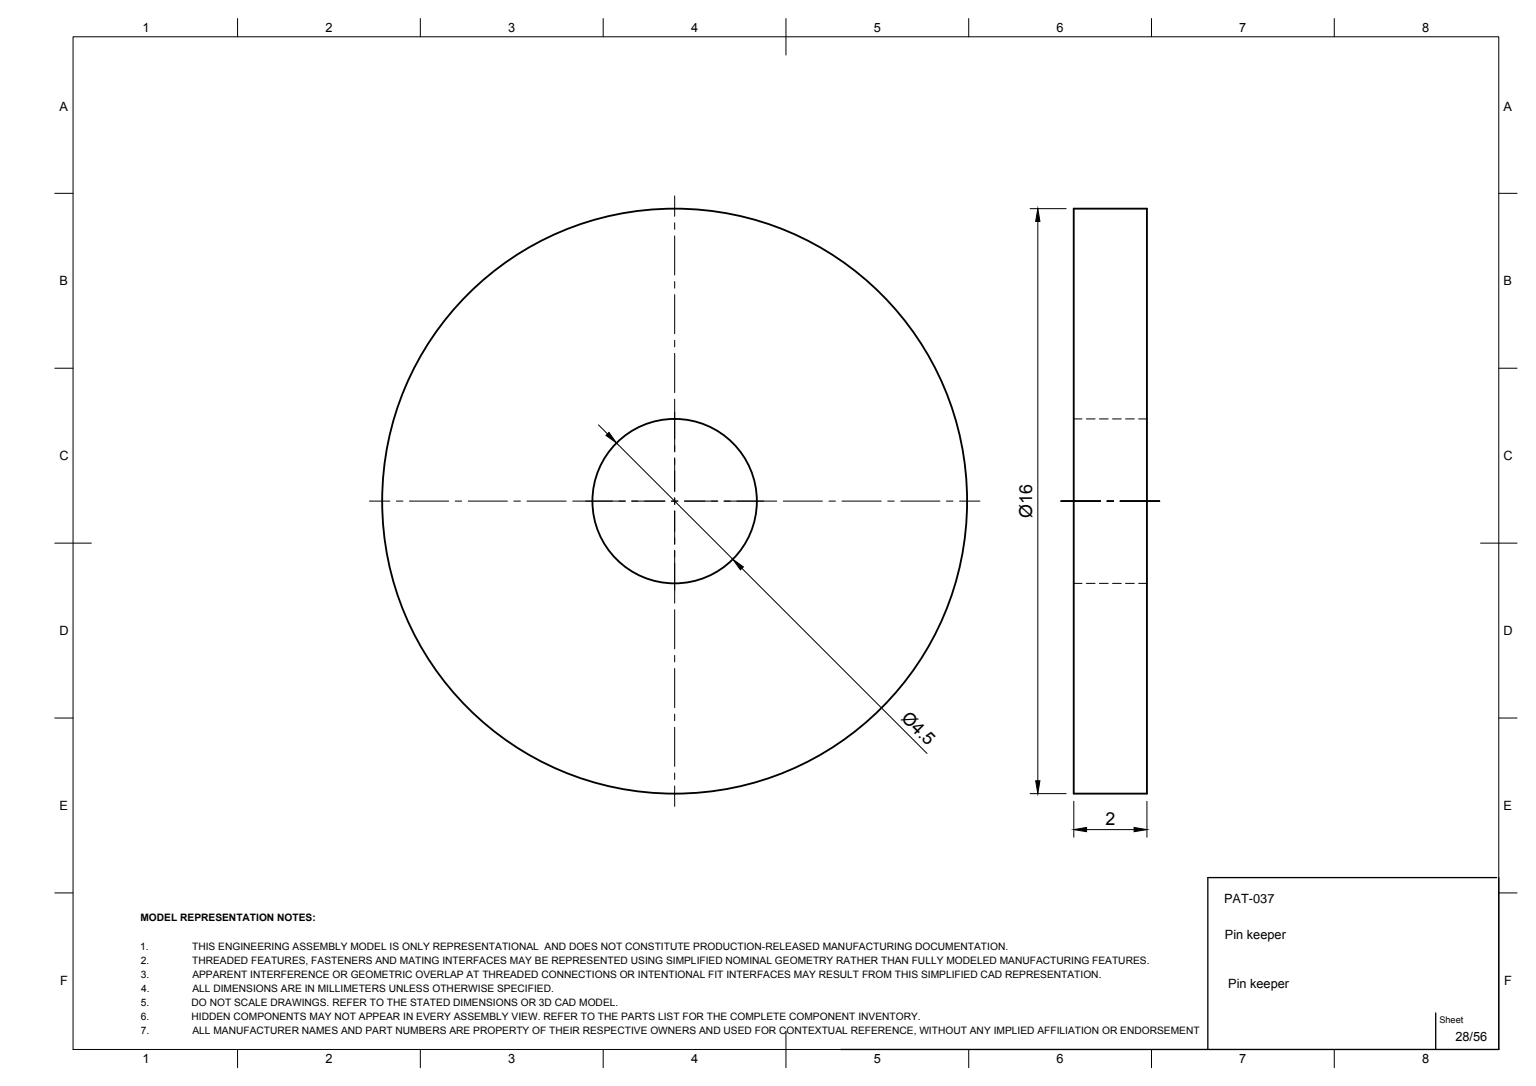
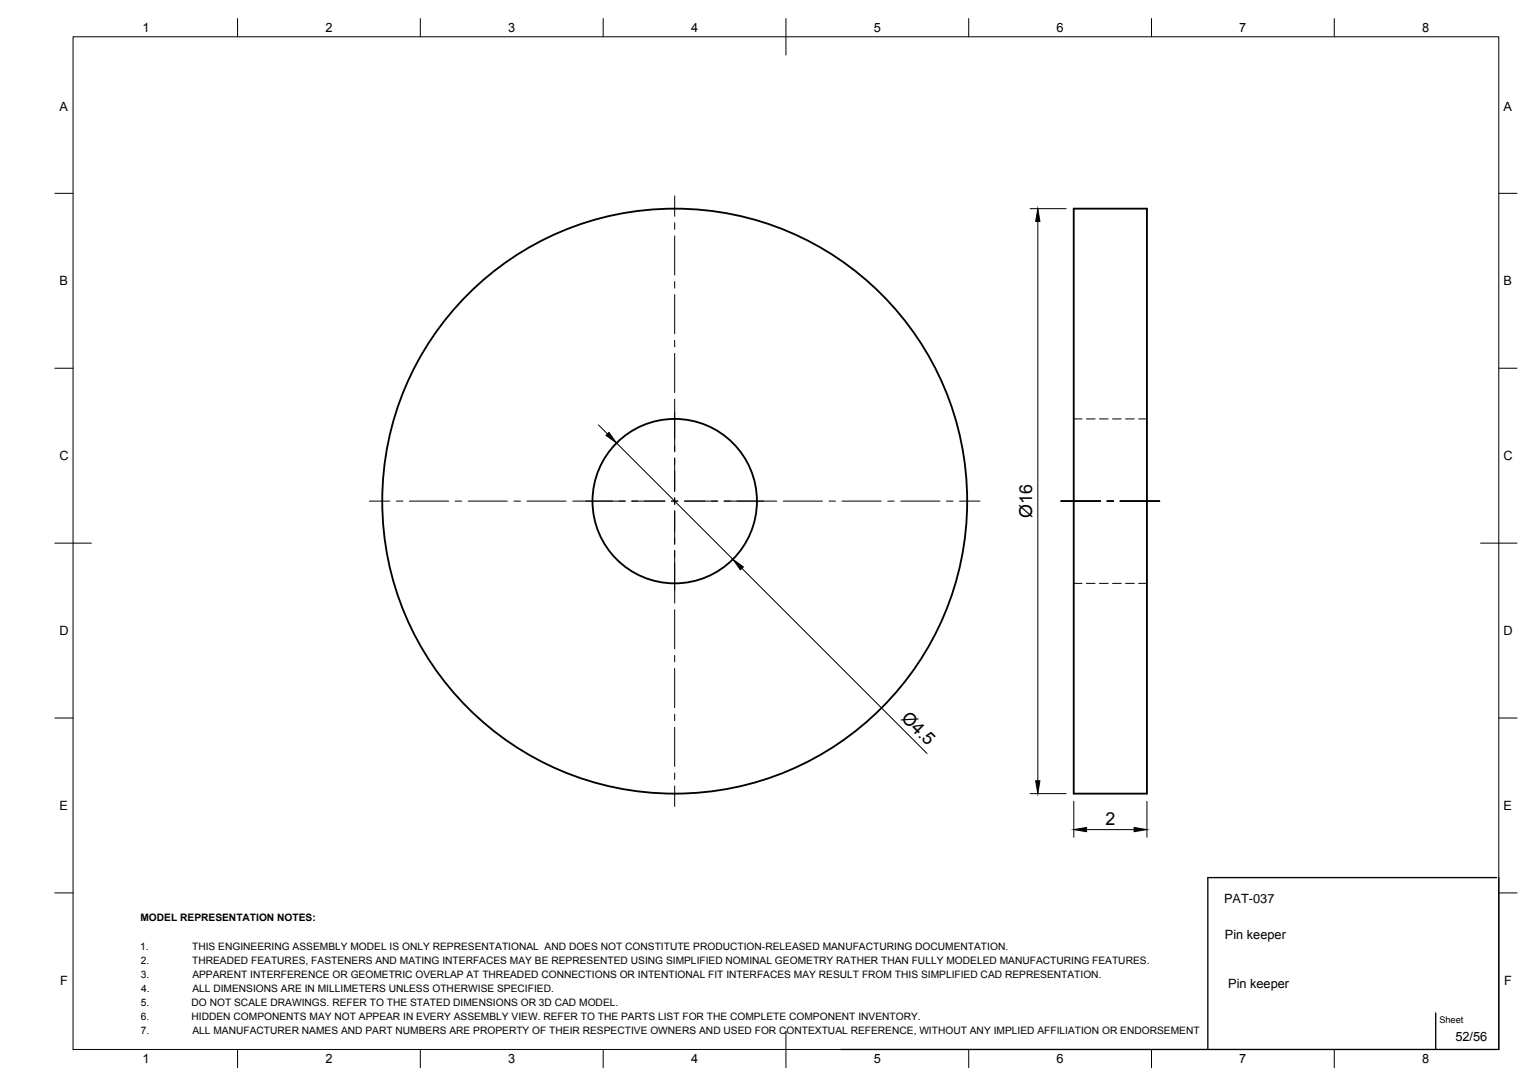
ISO-10303-21;
HEADER;
/* Generated by software containing ST-Developer
 * from STEP Tools, Inc. (www.steptools.com) 
 */

FILE_DESCRIPTION(
/* description */ ('Flywheel Crank-Slider'),
/* implementation_level */ '2;1');

FILE_NAME(
/* name */ 'Pin keeper.step',
/* time_stamp */ '2026-10-28T03:23:13-07:00',
/* author */ (''),
/* organization */ (''),
/* preprocessor_version */ 'ST-DEVELOPER v20.2',
/* originating_system */ 'Autodesk Translation Framework v15.17.0.0',
/* authorisation */ '');

FILE_SCHEMA (('AUTOMOTIVE_DESIGN { 1 0 10303 214 3 1 1 }'));
ENDSEC;

DATA;
#10=MECHANICAL_DESIGN_GEOMETRIC_PRESENTATION_REPRESENTATION('',(#698),#17322);
#593=SHAPE_REPRESENTATION_RELATIONSHIP('SRR','None',#17591,#645);
#645=ADVANCED_BREP_SHAPE_REPRESENTATION('',(#755),#17295);
#698=STYLED_ITEM('',(#17931),#755);
#755=MANIFOLD_SOLID_BREP('Body1',#9080);
#928=FACE_BOUND('',#2333,.T.);
#929=FACE_BOUND('',#2335,.T.);
#1209=PLANE('',#10309);
#1210=PLANE('',#10310);
#1652=FACE_OUTER_BOUND('',#2330,.T.);
#1653=FACE_OUTER_BOUND('',#2331,.T.);
#1654=FACE_OUTER_BOUND('',#2332,.T.);
#1655=FACE_OUTER_BOUND('',#2334,.T.);
#2330=EDGE_LOOP('',(#7504,#7505,#7506,#7507));
#2331=EDGE_LOOP('',(#7508,#7509,#7510,#7511));
#2332=EDGE_LOOP('',(#7512));
#2333=EDGE_LOOP('',(#7513));
#2334=EDGE_LOOP('',(#7514));
#2335=EDGE_LOOP('',(#7515));
#3021=LINE('',#15833,#3632);
#3022=LINE('',#15839,#3633);
#3632=VECTOR('',#12475,0.225);
#3633=VECTOR('',#12482,0.8);
#4088=CIRCLE('',#10304,0.225);
#4089=CIRCLE('',#10305,0.225);
#4090=CIRCLE('',#10307,0.8);
#4091=CIRCLE('',#10308,0.8);
#4735=VERTEX_POINT('',#15830);
#4736=VERTEX_POINT('',#15832);
#4737=VERTEX_POINT('',#15836);
#4738=VERTEX_POINT('',#15838);
#5709=EDGE_CURVE('',#4735,#4735,#4088,.T.);
#5710=EDGE_CURVE('',#4735,#4736,#3021,.T.);
#5711=EDGE_CURVE('',#4736,#4736,#4089,.T.);
#5712=EDGE_CURVE('',#4737,#4737,#4090,.T.);
#5713=EDGE_CURVE('',#4737,#4738,#3022,.T.);
#5714=EDGE_CURVE('',#4738,#4738,#4091,.T.);
#7504=ORIENTED_EDGE('',*,*,#5709,.F.);
#7505=ORIENTED_EDGE('',*,*,#5710,.T.);
#7506=ORIENTED_EDGE('',*,*,#5711,.T.);
#7507=ORIENTED_EDGE('',*,*,#5710,.F.);
#7508=ORIENTED_EDGE('',*,*,#5712,.F.);
#7509=ORIENTED_EDGE('',*,*,#5713,.T.);
#7510=ORIENTED_EDGE('',*,*,#5714,.T.);
#7511=ORIENTED_EDGE('',*,*,#5713,.F.);
#7512=ORIENTED_EDGE('',*,*,#5712,.T.);
#7513=ORIENTED_EDGE('',*,*,#5709,.T.);
#7514=ORIENTED_EDGE('',*,*,#5714,.F.);
#7515=ORIENTED_EDGE('',*,*,#5711,.F.);
#8446=CYLINDRICAL_SURFACE('',#10303,0.225);
#8447=CYLINDRICAL_SURFACE('',#10306,0.8);
#8843=ADVANCED_FACE('',(#1652),#8446,.F.);
#8844=ADVANCED_FACE('',(#1653),#8447,.T.);
#8845=ADVANCED_FACE('',(#1654,#928),#1209,.T.);
#8846=ADVANCED_FACE('',(#1655,#929),#1210,.F.);
#9080=CLOSED_SHELL('',(#8843,#8844,#8845,#8846));
#10302=AXIS2_PLACEMENT_3D('',#15828,#12469,#12470);
#10303=AXIS2_PLACEMENT_3D('',#15829,#12471,#12472);
#10304=AXIS2_PLACEMENT_3D('',#15831,#12473,#12474);
#10305=AXIS2_PLACEMENT_3D('',#15834,#12476,#12477);
#10306=AXIS2_PLACEMENT_3D('',#15835,#12478,#12479);
#10307=AXIS2_PLACEMENT_3D('',#15837,#12480,#12481);
#10308=AXIS2_PLACEMENT_3D('',#15840,#12483,#12484);
#10309=AXIS2_PLACEMENT_3D('',#15841,#12485,#12486);
#10310=AXIS2_PLACEMENT_3D('',#15842,#12487,#12488);
#12469=DIRECTION('axis',(0.,0.,1.));
#12470=DIRECTION('refdir',(1.,0.,0.));
#12471=DIRECTION('center_axis',(0.,1.,0.));
#12472=DIRECTION('ref_axis',(1.,0.,0.));
#12473=DIRECTION('center_axis',(0.,-1.,0.));
#12474=DIRECTION('ref_axis',(1.,0.,0.));
#12475=DIRECTION('',(0.,-1.,0.));
#12476=DIRECTION('center_axis',(0.,-1.,0.));
#12477=DIRECTION('ref_axis',(1.,0.,0.));
#12478=DIRECTION('center_axis',(0.,1.,0.));
#12479=DIRECTION('ref_axis',(1.,0.,0.));
#12480=DIRECTION('center_axis',(0.,1.,0.));
#12481=DIRECTION('ref_axis',(1.,0.,0.));
#12482=DIRECTION('',(0.,-1.,0.));
#12483=DIRECTION('center_axis',(0.,1.,0.));
#12484=DIRECTION('ref_axis',(1.,0.,0.));
#12485=DIRECTION('center_axis',(0.,1.,0.));
#12486=DIRECTION('ref_axis',(1.,0.,0.));
#12487=DIRECTION('center_axis',(0.,1.,0.));
#12488=DIRECTION('ref_axis',(1.,0.,0.));
#15828=CARTESIAN_POINT('',(0.,0.,0.));
#15829=CARTESIAN_POINT('Origin',(2.,3.8,10.));
#15830=CARTESIAN_POINT('',(1.775,4.,10.));
#15831=CARTESIAN_POINT('Origin',(2.,4.,10.));
#15832=CARTESIAN_POINT('',(1.775,3.8,10.));
#15833=CARTESIAN_POINT('',(1.775,3.8,10.));
#15834=CARTESIAN_POINT('Origin',(2.,3.8,10.));
#15835=CARTESIAN_POINT('Origin',(2.,3.8,10.));
#15836=CARTESIAN_POINT('',(1.2,4.,10.));
#15837=CARTESIAN_POINT('Origin',(2.,4.,10.));
#15838=CARTESIAN_POINT('',(1.2,3.8,10.));
#15839=CARTESIAN_POINT('',(1.2,3.8,10.));
#15840=CARTESIAN_POINT('Origin',(2.,3.8,10.));
#15841=CARTESIAN_POINT('Origin',(2.,4.,10.));
#15842=CARTESIAN_POINT('Origin',(2.,3.8,10.));
#17234=UNCERTAINTY_MEASURE_WITH_UNIT(LENGTH_MEASURE(0.001),#17323,
'DISTANCE_ACCURACY_VALUE',
'Maximum model space distance between geometric entities at asserted c
onnectivities');
#17261=UNCERTAINTY_MEASURE_WITH_UNIT(LENGTH_MEASURE(0.001),#17323,
'DISTANCE_ACCURACY_VALUE',
'Maximum model space distance between geometric entities at asserted c
onnectivities');
#17295=(
GEOMETRIC_REPRESENTATION_CONTEXT(3)
GLOBAL_UNCERTAINTY_ASSIGNED_CONTEXT((#17234))
GLOBAL_UNIT_ASSIGNED_CONTEXT((#17323,#17325,#17326))
REPRESENTATION_CONTEXT('','3D')
);
#17322=(
GEOMETRIC_REPRESENTATION_CONTEXT(3)
GLOBAL_UNCERTAINTY_ASSIGNED_CONTEXT((#17261))
GLOBAL_UNIT_ASSIGNED_CONTEXT((#17323,#17325,#17326))
REPRESENTATION_CONTEXT('','3D')
);
#17323=(
LENGTH_UNIT()
NAMED_UNIT(*)
SI_UNIT(.CENTI.,.METRE.)
);
#17325=(
NAMED_UNIT(*)
PLANE_ANGLE_UNIT()
SI_UNIT($,.RADIAN.)
);
#17326=(
NAMED_UNIT(*)
SI_UNIT($,.STERADIAN.)
SOLID_ANGLE_UNIT()
);
#17360=SHAPE_DEFINITION_REPRESENTATION(#17422,#17591);
#17422=PRODUCT_DEFINITION_SHAPE('',$,#17652);
#17591=SHAPE_REPRESENTATION('',(#10302),#17295);
#17618=PRODUCT_DEFINITION_CONTEXT('part definition',#17800,'design');
#17652=PRODUCT_DEFINITION('Pin keeper','Pin keeper',#17712,#17618);
#17712=PRODUCT_DEFINITION_FORMATION('',$,#17835);
#17800=APPLICATION_CONTEXT(
'Core Data for Automotive Mechanical Design Process');
#17801=PRODUCT_CONTEXT('part definition',#17800,'mechanical');
#17835=PRODUCT('Pin keeper','Pin keeper','Pin keeper',(#17801));
#17925=COLOUR_RGB('Grey',0.48,0.52,0.57);
#17926=FILL_AREA_STYLE_COLOUR('',#17925);
#17927=FILL_AREA_STYLE('',(#17926));
#17928=SURFACE_STYLE_FILL_AREA(#17927);
#17929=SURFACE_SIDE_STYLE('',(#17928));
#17930=SURFACE_STYLE_USAGE(.BOTH.,#17929);
#17931=PRESENTATION_STYLE_ASSIGNMENT((#17930));
ENDSEC;
END-ISO-10303-21;
